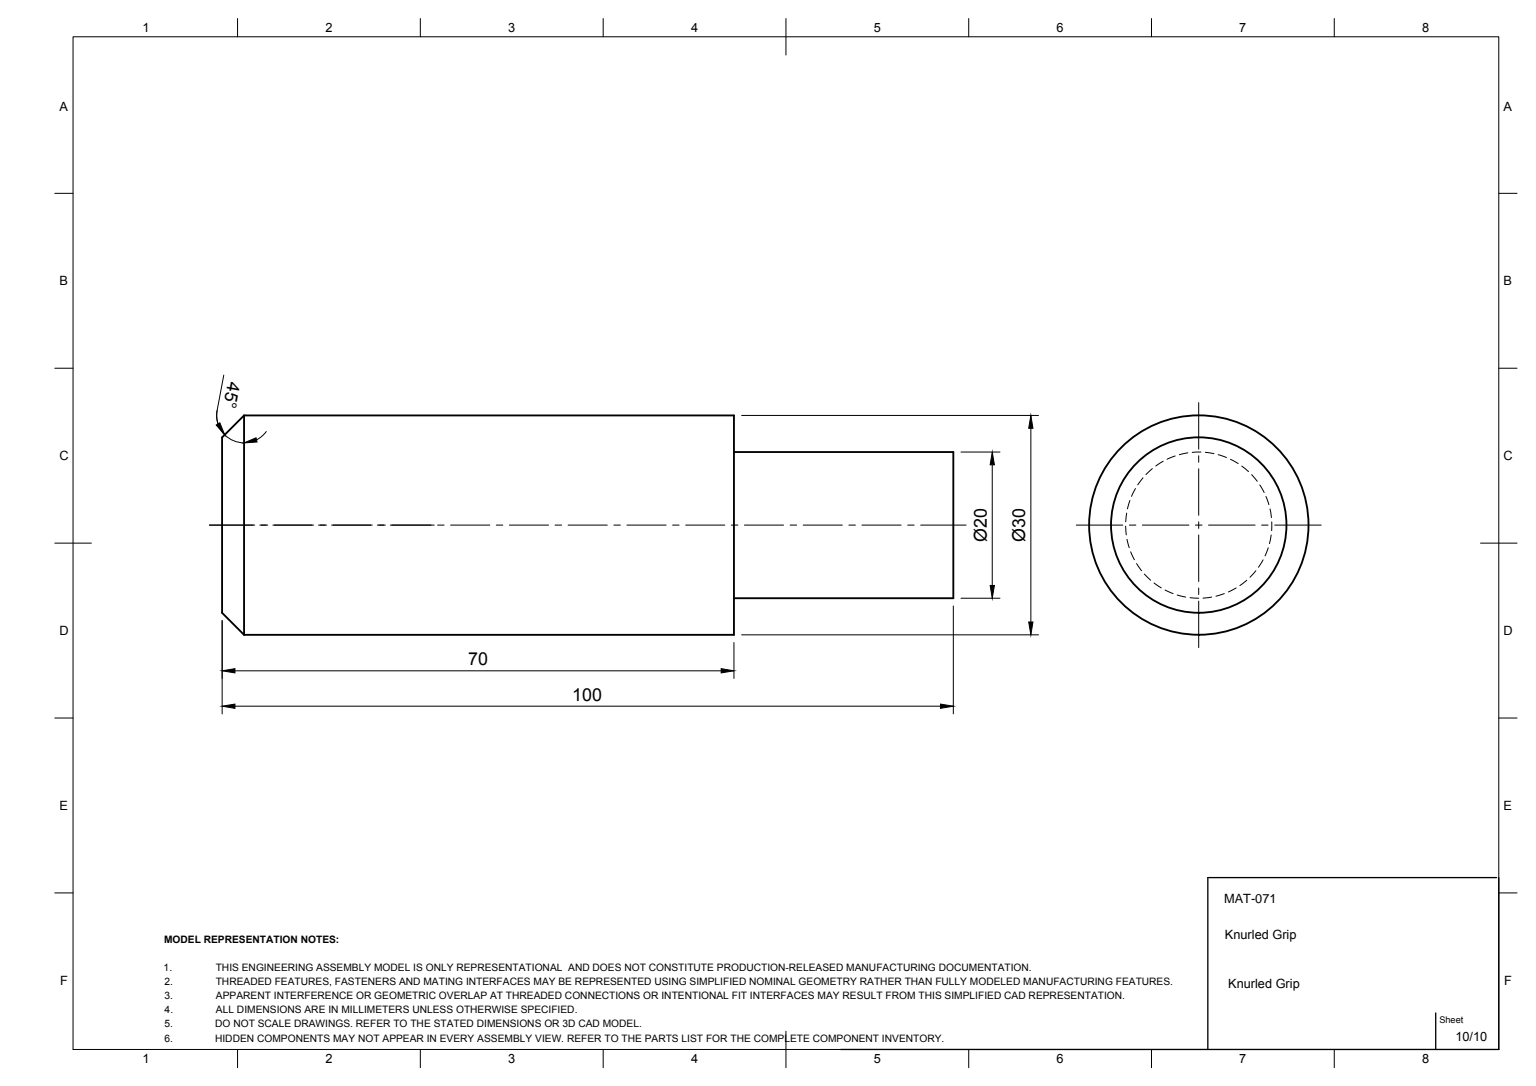
ISO-10303-21;
HEADER;
/* Generated by software containing ST-Developer
 * from STEP Tools, Inc. (www.steptools.com) 
 */

FILE_DESCRIPTION(
/* description */ (''),
/* implementation_level */ '2;1');

FILE_NAME(
/* name */ 'Knurled Grip.step',
/* time_stamp */ '2026-10-24T12:24:47-07:00',
/* author */ (''),
/* organization */ (''),
/* preprocessor_version */ 'ST-DEVELOPER v20.2',
/* originating_system */ 'Autodesk Translation Framework v15.15.0.0',
/* authorisation */ '');

FILE_SCHEMA (('AUTOMOTIVE_DESIGN { 1 0 10303 214 3 1 1 }'));
ENDSEC;

DATA;
#10=MECHANICAL_DESIGN_GEOMETRIC_PRESENTATION_REPRESENTATION('',(#58),#13594);
#46=SHAPE_REPRESENTATION_RELATIONSHIP('SRR','None',#13626,#52);
#52=ADVANCED_BREP_SHAPE_REPRESENTATION('',(#64),#13589);
#58=STYLED_ITEM('',(#13667),#64);
#64=MANIFOLD_SOLID_BREP('Knurled Grip',#2965);
#77=CONICAL_SURFACE('',#3178,15.,0.785398163397452);
#87=PLANE('',#3168);
#88=PLANE('',#3173);
#89=PLANE('',#3177);
#117=FACE_BOUND('',#502,.T.);
#161=CIRCLE('',#3169,12.);
#162=CIRCLE('',#3171,15.);
#163=CIRCLE('',#3172,15.);
#164=CIRCLE('',#3174,9.99999999999999);
#165=CIRCLE('',#3176,9.99999999999998);
#324=FACE_OUTER_BOUND('',#499,.T.);
#325=FACE_OUTER_BOUND('',#500,.T.);
#326=FACE_OUTER_BOUND('',#501,.T.);
#327=FACE_OUTER_BOUND('',#503,.T.);
#328=FACE_OUTER_BOUND('',#504,.T.);
#329=FACE_OUTER_BOUND('',#505,.T.);
#499=EDGE_LOOP('',(#2471));
#500=EDGE_LOOP('',(#2472,#2473,#2474,#2475));
#501=EDGE_LOOP('',(#2476));
#502=EDGE_LOOP('',(#2477));
#503=EDGE_LOOP('',(#2478,#2479,#2480,#2481));
#504=EDGE_LOOP('',(#2482));
#505=EDGE_LOOP('',(#2483,#2484,#2485,#2486));
#894=LINE('',#11059,#1045);
#895=LINE('',#11067,#1046);
#896=LINE('',#11070,#1047);
#1045=VECTOR('',#3660,15.);
#1046=VECTOR('',#3671,9.99999999999999);
#1047=VECTOR('',#3676,15.);
#1304=VERTEX_POINT('',#11053);
#1305=VERTEX_POINT('',#11056);
#1306=VERTEX_POINT('',#11058);
#1307=VERTEX_POINT('',#11062);
#1308=VERTEX_POINT('',#11065);
#1704=EDGE_CURVE('',#1304,#1304,#161,.F.);
#1705=EDGE_CURVE('',#1305,#1305,#162,.T.);
#1706=EDGE_CURVE('',#1305,#1306,#894,.T.);
#1707=EDGE_CURVE('',#1306,#1306,#163,.T.);
#1708=EDGE_CURVE('',#1307,#1307,#164,.T.);
#1709=EDGE_CURVE('',#1308,#1308,#165,.T.);
#1710=EDGE_CURVE('',#1308,#1307,#895,.T.);
#1711=EDGE_CURVE('',#1306,#1304,#896,.T.);
#2471=ORIENTED_EDGE('',*,*,#1704,.T.);
#2472=ORIENTED_EDGE('',*,*,#1705,.F.);
#2473=ORIENTED_EDGE('',*,*,#1706,.T.);
#2474=ORIENTED_EDGE('',*,*,#1707,.T.);
#2475=ORIENTED_EDGE('',*,*,#1706,.F.);
#2476=ORIENTED_EDGE('',*,*,#1705,.T.);
#2477=ORIENTED_EDGE('',*,*,#1708,.F.);
#2478=ORIENTED_EDGE('',*,*,#1709,.F.);
#2479=ORIENTED_EDGE('',*,*,#1710,.T.);
#2480=ORIENTED_EDGE('',*,*,#1708,.T.);
#2481=ORIENTED_EDGE('',*,*,#1710,.F.);
#2482=ORIENTED_EDGE('',*,*,#1709,.T.);
#2483=ORIENTED_EDGE('',*,*,#1707,.F.);
#2484=ORIENTED_EDGE('',*,*,#1711,.T.);
#2485=ORIENTED_EDGE('',*,*,#1704,.F.);
#2486=ORIENTED_EDGE('',*,*,#1711,.F.);
#2774=CYLINDRICAL_SURFACE('',#3170,15.);
#2775=CYLINDRICAL_SURFACE('',#3175,9.99999999999999);
#2911=ADVANCED_FACE('',(#324),#87,.F.);
#2912=ADVANCED_FACE('',(#325),#2774,.T.);
#2913=ADVANCED_FACE('',(#326,#117),#88,.F.);
#2914=ADVANCED_FACE('',(#327),#2775,.T.);
#2915=ADVANCED_FACE('',(#328),#89,.F.);
#2916=ADVANCED_FACE('',(#329),#77,.T.);
#2965=CLOSED_SHELL('',(#2911,#2912,#2913,#2914,#2915,#2916));
#3167=AXIS2_PLACEMENT_3D('',#11051,#3650,#3651);
#3168=AXIS2_PLACEMENT_3D('',#11052,#3652,#3653);
#3169=AXIS2_PLACEMENT_3D('',#11054,#3654,#3655);
#3170=AXIS2_PLACEMENT_3D('',#11055,#3656,#3657);
#3171=AXIS2_PLACEMENT_3D('',#11057,#3658,#3659);
#3172=AXIS2_PLACEMENT_3D('',#11060,#3661,#3662);
#3173=AXIS2_PLACEMENT_3D('',#11061,#3663,#3664);
#3174=AXIS2_PLACEMENT_3D('',#11063,#3665,#3666);
#3175=AXIS2_PLACEMENT_3D('',#11064,#3667,#3668);
#3176=AXIS2_PLACEMENT_3D('',#11066,#3669,#3670);
#3177=AXIS2_PLACEMENT_3D('',#11068,#3672,#3673);
#3178=AXIS2_PLACEMENT_3D('',#11069,#3674,#3675);
#3650=DIRECTION('axis',(0.,0.,1.));
#3651=DIRECTION('refdir',(1.,0.,0.));
#3652=DIRECTION('center_axis',(-1.,0.,0.));
#3653=DIRECTION('ref_axis',(0.,0.,1.));
#3654=DIRECTION('center_axis',(-1.,0.,0.));
#3655=DIRECTION('ref_axis',(0.,0.,1.));
#3656=DIRECTION('center_axis',(-1.,0.,0.));
#3657=DIRECTION('ref_axis',(0.,0.,1.));
#3658=DIRECTION('center_axis',(-1.,0.,0.));
#3659=DIRECTION('ref_axis',(0.,0.,1.));
#3660=DIRECTION('',(1.,0.,0.));
#3661=DIRECTION('center_axis',(-1.,0.,0.));
#3662=DIRECTION('ref_axis',(0.,0.,1.));
#3663=DIRECTION('center_axis',(1.,0.,0.));
#3664=DIRECTION('ref_axis',(0.,0.,-1.));
#3665=DIRECTION('center_axis',(-1.,0.,0.));
#3666=DIRECTION('ref_axis',(0.,0.,1.));
#3667=DIRECTION('center_axis',(-1.,0.,0.));
#3668=DIRECTION('ref_axis',(0.,0.,1.));
#3669=DIRECTION('center_axis',(-1.,0.,0.));
#3670=DIRECTION('ref_axis',(0.,0.,1.));
#3671=DIRECTION('',(1.,0.,0.));
#3672=DIRECTION('center_axis',(1.,0.,0.));
#3673=DIRECTION('ref_axis',(0.,0.,-1.));
#3674=DIRECTION('center_axis',(-1.,0.,0.));
#3675=DIRECTION('ref_axis',(0.,0.,1.));
#3676=DIRECTION('',(0.707106781186545,8.65956056235497E-17,0.70710678118655));
#11051=CARTESIAN_POINT('',(0.,0.,0.));
#11052=CARTESIAN_POINT('Origin',(215.,50.,0.));
#11053=CARTESIAN_POINT('',(215.,50.,-12.));
#11054=CARTESIAN_POINT('Origin',(215.,50.,0.));
#11055=CARTESIAN_POINT('Origin',(-266.943789971923,50.,0.));
#11056=CARTESIAN_POINT('',(145.,50.,-15.));
#11057=CARTESIAN_POINT('Origin',(145.,50.,0.));
#11058=CARTESIAN_POINT('',(212.,50.,-15.));
#11059=CARTESIAN_POINT('',(-266.943789971923,50.,-15.));
#11060=CARTESIAN_POINT('Origin',(212.,50.,0.));
#11061=CARTESIAN_POINT('Origin',(145.,50.,-15.));
#11062=CARTESIAN_POINT('',(145.,50.,-9.99999999999999));
#11063=CARTESIAN_POINT('Origin',(145.,50.,0.));
#11064=CARTESIAN_POINT('Origin',(-266.943789971923,50.,0.));
#11065=CARTESIAN_POINT('',(115.,50.,-9.99999999999999));
#11066=CARTESIAN_POINT('Origin',(115.,50.,0.));
#11067=CARTESIAN_POINT('',(-266.943789971923,50.,-9.99999999999999));
#11068=CARTESIAN_POINT('Origin',(115.,50.,-9.99999999999998));
#11069=CARTESIAN_POINT('Origin',(212.,50.,0.));
#11070=CARTESIAN_POINT('',(212.,50.,-15.));
#13580=UNCERTAINTY_MEASURE_WITH_UNIT(LENGTH_MEASURE(0.01),#13595,
'DISTANCE_ACCURACY_VALUE',
'Maximum model space distance between geometric entities at asserted c
onnectivities');
#13585=UNCERTAINTY_MEASURE_WITH_UNIT(LENGTH_MEASURE(0.01),#13595,
'DISTANCE_ACCURACY_VALUE',
'Maximum model space distance between geometric entities at asserted c
onnectivities');
#13589=(
GEOMETRIC_REPRESENTATION_CONTEXT(3)
GLOBAL_UNCERTAINTY_ASSIGNED_CONTEXT((#13580))
GLOBAL_UNIT_ASSIGNED_CONTEXT((#13595,#13597,#13598))
REPRESENTATION_CONTEXT('','3D')
);
#13594=(
GEOMETRIC_REPRESENTATION_CONTEXT(3)
GLOBAL_UNCERTAINTY_ASSIGNED_CONTEXT((#13585))
GLOBAL_UNIT_ASSIGNED_CONTEXT((#13595,#13597,#13598))
REPRESENTATION_CONTEXT('','3D')
);
#13595=(
LENGTH_UNIT()
NAMED_UNIT(*)
SI_UNIT(.MILLI.,.METRE.)
);
#13597=(
NAMED_UNIT(*)
PLANE_ANGLE_UNIT()
SI_UNIT($,.RADIAN.)
);
#13598=(
NAMED_UNIT(*)
SI_UNIT($,.STERADIAN.)
SOLID_ANGLE_UNIT()
);
#13602=SHAPE_DEFINITION_REPRESENTATION(#13610,#13626);
#13610=PRODUCT_DEFINITION_SHAPE('',$,#13635);
#13626=SHAPE_REPRESENTATION('',(#3167),#13589);
#13631=PRODUCT_DEFINITION_CONTEXT('part definition',#13657,'design');
#13635=PRODUCT_DEFINITION('Knurled Grip','Knurled Grip',#13643,#13631);
#13643=PRODUCT_DEFINITION_FORMATION('',$,#13662);
#13657=APPLICATION_CONTEXT(
'Core Data for Automotive Mechanical Design Process');
#13658=PRODUCT_CONTEXT('part definition',#13657,'mechanical');
#13662=PRODUCT('Knurled Grip','Knurled Grip',$,(#13658));
#13667=PRESENTATION_STYLE_ASSIGNMENT((#13668));
#13668=SURFACE_STYLE_USAGE(.BOTH.,#13669);
#13669=SURFACE_SIDE_STYLE('',(#13670));
#13670=SURFACE_STYLE_FILL_AREA(#13671);
#13671=FILL_AREA_STYLE('Steel - Satin',(#13672));
#13672=FILL_AREA_STYLE_COLOUR('Steel - Satin',#13673);
#13673=COLOUR_RGB('Steel - Satin',0.627450980392157,0.627450980392157,0.627450980392157);
ENDSEC;
END-ISO-10303-21;
